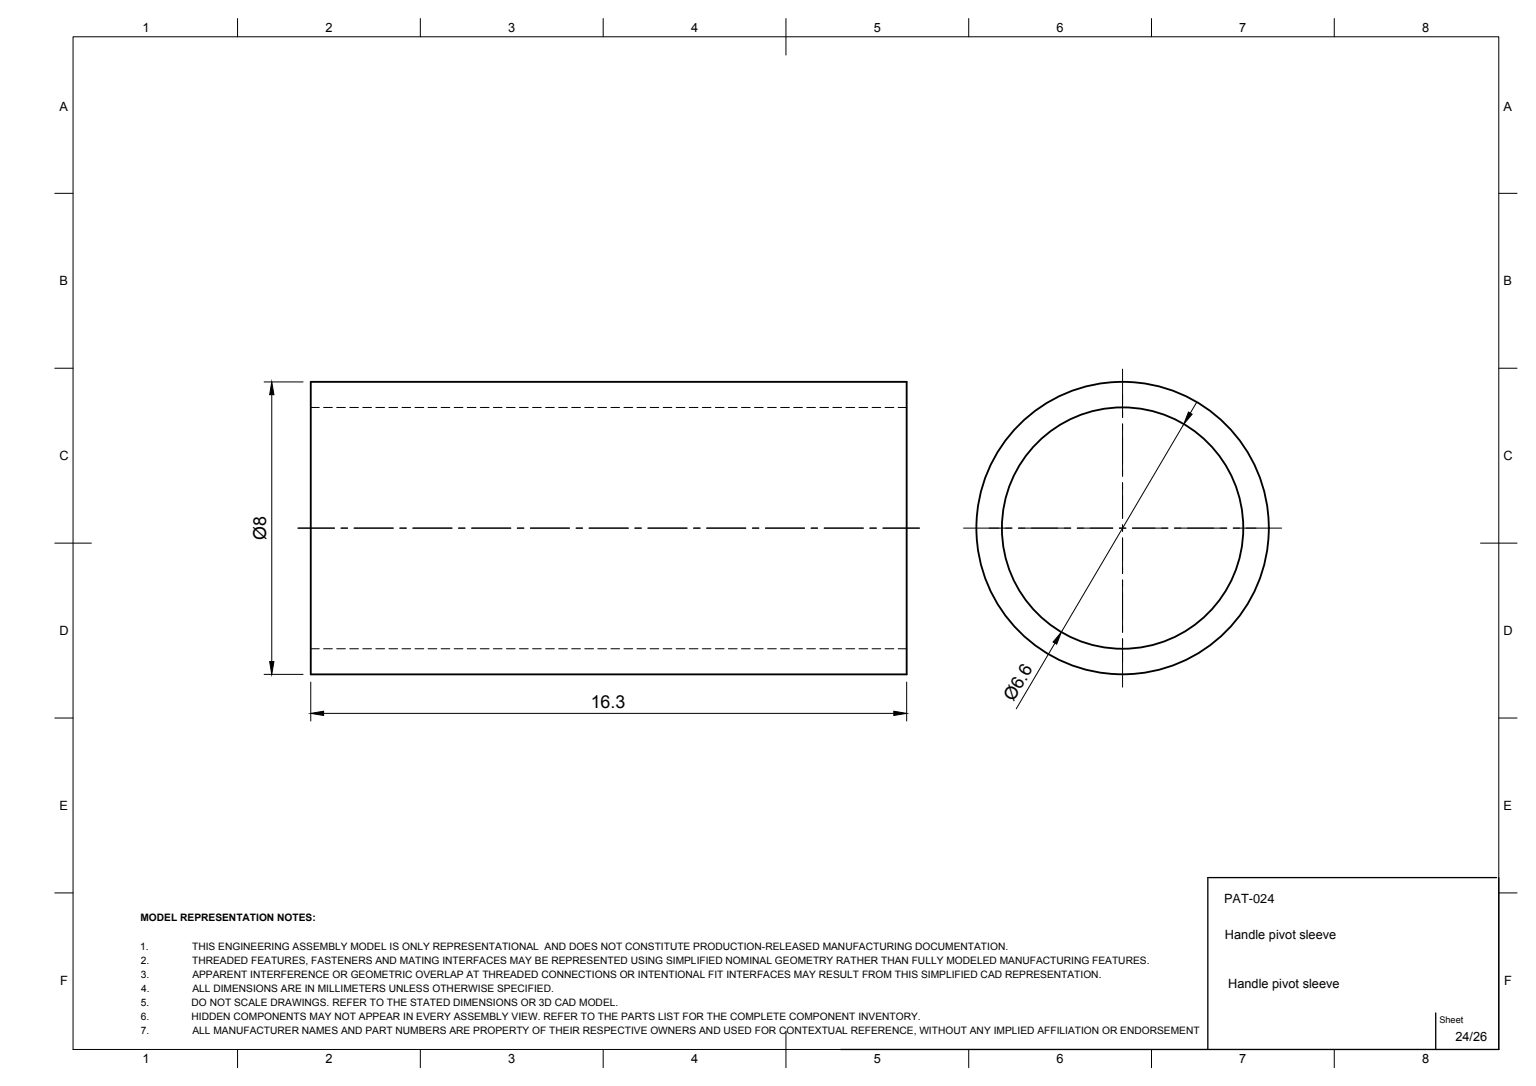
ISO-10303-21;
HEADER;
/* Generated by software containing ST-Developer
 * from STEP Tools, Inc. (www.steptools.com) 
 */

FILE_DESCRIPTION(
/* description */ ('Compact handwheel screw vise'),
/* implementation_level */ '2;1');

FILE_NAME(
/* name */ 'Handle pivot sleeve.step',
/* time_stamp */ '2026-10-29T16:08:22-07:00',
/* author */ (''),
/* organization */ (''),
/* preprocessor_version */ 'ST-DEVELOPER v20.2',
/* originating_system */ 'Autodesk Translation Framework v15.17.0.0',
/* authorisation */ '');

FILE_SCHEMA (('AUTOMOTIVE_DESIGN { 1 0 10303 214 3 1 1 }'));
ENDSEC;

DATA;
#10=MECHANICAL_DESIGN_GEOMETRIC_PRESENTATION_REPRESENTATION('',(#674),#25074);
#610=SHAPE_REPRESENTATION_RELATIONSHIP('SRR','None',#25221,#638);
#638=ADVANCED_BREP_SHAPE_REPRESENTATION('',(#707),#25068);
#674=STYLED_ITEM('',(#25432),#707);
#707=MANIFOLD_SOLID_BREP('Body1',#8085);
#814=FACE_BOUND('',#2006,.T.);
#815=FACE_BOUND('',#2008,.T.);
#976=PLANE('',#9097);
#977=PLANE('',#9098);
#1431=FACE_OUTER_BOUND('',#2003,.T.);
#1432=FACE_OUTER_BOUND('',#2004,.T.);
#1433=FACE_OUTER_BOUND('',#2005,.T.);
#1434=FACE_OUTER_BOUND('',#2007,.T.);
#2003=EDGE_LOOP('',(#7147,#7148,#7149,#7150));
#2004=EDGE_LOOP('',(#7151,#7152,#7153,#7154));
#2005=EDGE_LOOP('',(#7155));
#2006=EDGE_LOOP('',(#7156));
#2007=EDGE_LOOP('',(#7157));
#2008=EDGE_LOOP('',(#7158));
#2495=LINE('',#24759,#3003);
#2496=LINE('',#24765,#3004);
#3003=VECTOR('',#11021,0.33);
#3004=VECTOR('',#11028,0.4);
#3309=CIRCLE('',#9092,0.33);
#3310=CIRCLE('',#9093,0.33);
#3311=CIRCLE('',#9095,0.4);
#3312=CIRCLE('',#9096,0.4);
#4002=VERTEX_POINT('',#24756);
#4003=VERTEX_POINT('',#24758);
#4004=VERTEX_POINT('',#24762);
#4005=VERTEX_POINT('',#24764);
#5060=EDGE_CURVE('',#4002,#4002,#3309,.T.);
#5061=EDGE_CURVE('',#4002,#4003,#2495,.T.);
#5062=EDGE_CURVE('',#4003,#4003,#3310,.T.);
#5063=EDGE_CURVE('',#4004,#4004,#3311,.T.);
#5064=EDGE_CURVE('',#4004,#4005,#2496,.T.);
#5065=EDGE_CURVE('',#4005,#4005,#3312,.T.);
#7147=ORIENTED_EDGE('',*,*,#5060,.F.);
#7148=ORIENTED_EDGE('',*,*,#5061,.T.);
#7149=ORIENTED_EDGE('',*,*,#5062,.T.);
#7150=ORIENTED_EDGE('',*,*,#5061,.F.);
#7151=ORIENTED_EDGE('',*,*,#5063,.F.);
#7152=ORIENTED_EDGE('',*,*,#5064,.T.);
#7153=ORIENTED_EDGE('',*,*,#5065,.T.);
#7154=ORIENTED_EDGE('',*,*,#5064,.F.);
#7155=ORIENTED_EDGE('',*,*,#5063,.T.);
#7156=ORIENTED_EDGE('',*,*,#5060,.T.);
#7157=ORIENTED_EDGE('',*,*,#5065,.F.);
#7158=ORIENTED_EDGE('',*,*,#5062,.F.);
#7573=CYLINDRICAL_SURFACE('',#9091,0.33);
#7574=CYLINDRICAL_SURFACE('',#9094,0.4);
#8001=ADVANCED_FACE('',(#1431),#7573,.F.);
#8002=ADVANCED_FACE('',(#1432),#7574,.T.);
#8003=ADVANCED_FACE('',(#1433,#814),#976,.T.);
#8004=ADVANCED_FACE('',(#1434,#815),#977,.F.);
#8085=CLOSED_SHELL('',(#8001,#8002,#8003,#8004));
#9090=AXIS2_PLACEMENT_3D('',#24754,#11015,#11016);
#9091=AXIS2_PLACEMENT_3D('',#24755,#11017,#11018);
#9092=AXIS2_PLACEMENT_3D('',#24757,#11019,#11020);
#9093=AXIS2_PLACEMENT_3D('',#24760,#11022,#11023);
#9094=AXIS2_PLACEMENT_3D('',#24761,#11024,#11025);
#9095=AXIS2_PLACEMENT_3D('',#24763,#11026,#11027);
#9096=AXIS2_PLACEMENT_3D('',#24766,#11029,#11030);
#9097=AXIS2_PLACEMENT_3D('',#24767,#11031,#11032);
#9098=AXIS2_PLACEMENT_3D('',#24768,#11033,#11034);
#11015=DIRECTION('axis',(0.,0.,1.));
#11016=DIRECTION('refdir',(1.,0.,0.));
#11017=DIRECTION('center_axis',(1.,0.,0.));
#11018=DIRECTION('ref_axis',(0.,0.,-1.));
#11019=DIRECTION('center_axis',(-1.,0.,0.));
#11020=DIRECTION('ref_axis',(0.,0.,-1.));
#11021=DIRECTION('',(-1.,0.,0.));
#11022=DIRECTION('center_axis',(-1.,0.,0.));
#11023=DIRECTION('ref_axis',(0.,0.,-1.));
#11024=DIRECTION('center_axis',(1.,0.,0.));
#11025=DIRECTION('ref_axis',(0.,0.,-1.));
#11026=DIRECTION('center_axis',(1.,0.,0.));
#11027=DIRECTION('ref_axis',(0.,0.,-1.));
#11028=DIRECTION('',(-1.,0.,0.));
#11029=DIRECTION('center_axis',(1.,0.,0.));
#11030=DIRECTION('ref_axis',(0.,0.,-1.));
#11031=DIRECTION('center_axis',(1.,0.,0.));
#11032=DIRECTION('ref_axis',(0.,0.,-1.));
#11033=DIRECTION('center_axis',(1.,0.,0.));
#11034=DIRECTION('ref_axis',(0.,0.,-1.));
#24754=CARTESIAN_POINT('',(0.,0.,0.));
#24755=CARTESIAN_POINT('Origin',(29.4,0.,6.5));
#24756=CARTESIAN_POINT('',(31.03,-4.04133443718627E-17,6.83));
#24757=CARTESIAN_POINT('Origin',(31.03,0.,6.5));
#24758=CARTESIAN_POINT('',(29.4,-4.04133443718627E-17,6.83));
#24759=CARTESIAN_POINT('',(29.4,-4.04133443718627E-17,6.83));
#24760=CARTESIAN_POINT('Origin',(29.4,0.,6.5));
#24761=CARTESIAN_POINT('Origin',(29.4,0.,6.5));
#24762=CARTESIAN_POINT('',(31.03,-4.89858719658942E-17,6.9));
#24763=CARTESIAN_POINT('Origin',(31.03,0.,6.5));
#24764=CARTESIAN_POINT('',(29.4,-4.89858719658942E-17,6.9));
#24765=CARTESIAN_POINT('',(29.4,-4.89858719658942E-17,6.9));
#24766=CARTESIAN_POINT('Origin',(29.4,0.,6.5));
#24767=CARTESIAN_POINT('Origin',(31.03,0.,6.5));
#24768=CARTESIAN_POINT('Origin',(29.4,0.,6.5));
#25034=UNCERTAINTY_MEASURE_WITH_UNIT(LENGTH_MEASURE(0.001),#25075,
'DISTANCE_ACCURACY_VALUE',
'Maximum model space distance between geometric entities at asserted c
onnectivities');
#25040=UNCERTAINTY_MEASURE_WITH_UNIT(LENGTH_MEASURE(0.001),#25075,
'DISTANCE_ACCURACY_VALUE',
'Maximum model space distance between geometric entities at asserted c
onnectivities');
#25068=(
GEOMETRIC_REPRESENTATION_CONTEXT(3)
GLOBAL_UNCERTAINTY_ASSIGNED_CONTEXT((#25034))
GLOBAL_UNIT_ASSIGNED_CONTEXT((#25075,#25077,#25078))
REPRESENTATION_CONTEXT('','3D')
);
#25074=(
GEOMETRIC_REPRESENTATION_CONTEXT(3)
GLOBAL_UNCERTAINTY_ASSIGNED_CONTEXT((#25040))
GLOBAL_UNIT_ASSIGNED_CONTEXT((#25075,#25077,#25078))
REPRESENTATION_CONTEXT('','3D')
);
#25075=(
LENGTH_UNIT()
NAMED_UNIT(*)
SI_UNIT(.CENTI.,.METRE.)
);
#25077=(
NAMED_UNIT(*)
PLANE_ANGLE_UNIT()
SI_UNIT($,.RADIAN.)
);
#25078=(
NAMED_UNIT(*)
SI_UNIT($,.STERADIAN.)
SOLID_ANGLE_UNIT()
);
#25106=SHAPE_DEFINITION_REPRESENTATION(#25155,#25221);
#25155=PRODUCT_DEFINITION_SHAPE('',$,#25255);
#25221=SHAPE_REPRESENTATION('',(#9090),#25068);
#25227=PRODUCT_DEFINITION_CONTEXT('part definition',#25328,'design');
#25255=PRODUCT_DEFINITION('Handle pivot sleeve','Handle pivot sleeve',#25288,
#25227);
#25288=PRODUCT_DEFINITION_FORMATION('',$,#25357);
#25328=APPLICATION_CONTEXT(
'Core Data for Automotive Mechanical Design Process');
#25329=PRODUCT_CONTEXT('part definition',#25328,'mechanical');
#25357=PRODUCT('Handle pivot sleeve','Handle pivot sleeve',
'Handle pivot sleeve',(#25329));
#25426=COLOUR_RGB('Sky Blue',0.24,0.69,0.87);
#25427=FILL_AREA_STYLE_COLOUR('',#25426);
#25428=FILL_AREA_STYLE('',(#25427));
#25429=SURFACE_STYLE_FILL_AREA(#25428);
#25430=SURFACE_SIDE_STYLE('',(#25429));
#25431=SURFACE_STYLE_USAGE(.BOTH.,#25430);
#25432=PRESENTATION_STYLE_ASSIGNMENT((#25431));
ENDSEC;
END-ISO-10303-21;
